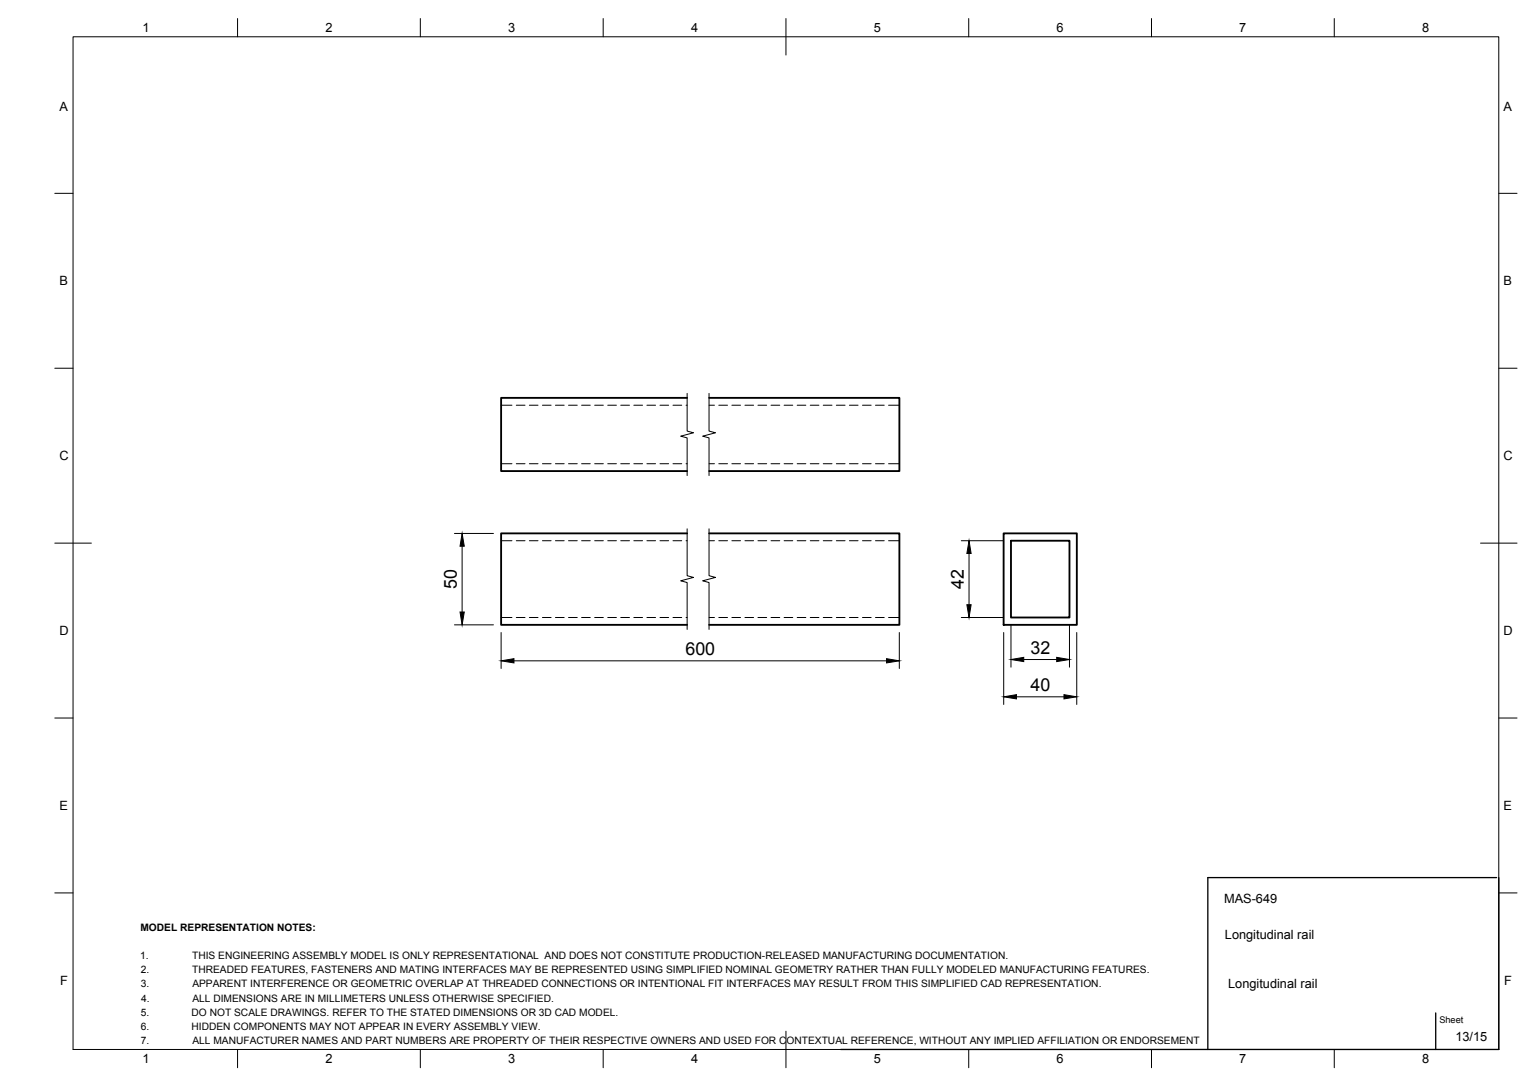
ISO-10303-21;
HEADER;
/* Generated by software containing ST-Developer
 * from STEP Tools, Inc. (www.steptools.com) 
 */

FILE_DESCRIPTION(
/* description */ ('Independent equipment support assembly with bolted 600 x 500 mm welde
d perimeter frame, four adjustable legs and swivel feet. Nominal overa
ll height 518 mm. No load rating assigned.'),
/* implementation_level */ '2;1');

FILE_NAME(
/* name */ 'Longitudinal rail.step',
/* time_stamp */ '2026-11-07T17:30:39-08:00',
/* author */ (''),
/* organization */ (''),
/* preprocessor_version */ 'ST-DEVELOPER v20.2',
/* originating_system */ 'Autodesk Translation Framework v15.17.0.0',
/* authorisation */ '');

FILE_SCHEMA (('AUTOMOTIVE_DESIGN { 1 0 10303 214 3 1 1 }'));
ENDSEC;

DATA;
#10=MECHANICAL_DESIGN_GEOMETRIC_PRESENTATION_REPRESENTATION('',(#2208),#63755);
#2176=SHAPE_REPRESENTATION_RELATIONSHIP('SRR','None',#63860,#2192);
#2192=ADVANCED_BREP_SHAPE_REPRESENTATION('',(#2224),#63738);
#2208=STYLED_ITEM('',(#63958),#2224);
#2224=MANIFOLD_SOLID_BREP('Body1',#14309);
#2240=FACE_BOUND('',#3072,.T.);
#2241=FACE_BOUND('',#3074,.T.);
#2303=FACE_OUTER_BOUND('',#3063,.T.);
#2304=FACE_OUTER_BOUND('',#3064,.T.);
#2305=FACE_OUTER_BOUND('',#3065,.T.);
#2306=FACE_OUTER_BOUND('',#3066,.T.);
#2307=FACE_OUTER_BOUND('',#3067,.T.);
#2308=FACE_OUTER_BOUND('',#3068,.T.);
#2309=FACE_OUTER_BOUND('',#3069,.T.);
#2310=FACE_OUTER_BOUND('',#3070,.T.);
#2311=FACE_OUTER_BOUND('',#3071,.T.);
#2312=FACE_OUTER_BOUND('',#3073,.T.);
#3063=EDGE_LOOP('',(#9127,#9128,#9129,#9130));
#3064=EDGE_LOOP('',(#9131,#9132,#9133,#9134));
#3065=EDGE_LOOP('',(#9135,#9136,#9137,#9138));
#3066=EDGE_LOOP('',(#9139,#9140,#9141,#9142));
#3067=EDGE_LOOP('',(#9143,#9144,#9145,#9146));
#3068=EDGE_LOOP('',(#9147,#9148,#9149,#9150));
#3069=EDGE_LOOP('',(#9151,#9152,#9153,#9154));
#3070=EDGE_LOOP('',(#9155,#9156,#9157,#9158));
#3071=EDGE_LOOP('',(#9159,#9160,#9161,#9162));
#3072=EDGE_LOOP('',(#9163,#9164,#9165,#9166));
#3073=EDGE_LOOP('',(#9167,#9168,#9169,#9170));
#3074=EDGE_LOOP('',(#9171,#9172,#9173,#9174));
#3886=LINE('',#18383,#4722);
#3887=LINE('',#18385,#4723);
#3888=LINE('',#18387,#4724);
#3889=LINE('',#18388,#4725);
#3890=LINE('',#18391,#4726);
#3891=LINE('',#18393,#4727);
#3892=LINE('',#18394,#4728);
#3893=LINE('',#18397,#4729);
#3894=LINE('',#18399,#4730);
#3895=LINE('',#18400,#4731);
#3896=LINE('',#18402,#4732);
#3897=LINE('',#18403,#4733);
#3898=LINE('',#18407,#4734);
#3899=LINE('',#18409,#4735);
#3900=LINE('',#18411,#4736);
#3901=LINE('',#18412,#4737);
#3902=LINE('',#18415,#4738);
#3903=LINE('',#18417,#4739);
#3904=LINE('',#18418,#4740);
#3905=LINE('',#18421,#4741);
#3906=LINE('',#18423,#4742);
#3907=LINE('',#18424,#4743);
#3908=LINE('',#18426,#4744);
#3909=LINE('',#18427,#4745);
#4722=VECTOR('',#15523,10.);
#4723=VECTOR('',#15524,10.);
#4724=VECTOR('',#15525,10.);
#4725=VECTOR('',#15526,10.);
#4726=VECTOR('',#15529,10.);
#4727=VECTOR('',#15530,10.);
#4728=VECTOR('',#15531,10.);
#4729=VECTOR('',#15534,10.);
#4730=VECTOR('',#15535,10.);
#4731=VECTOR('',#15536,10.);
#4732=VECTOR('',#15539,10.);
#4733=VECTOR('',#15540,10.);
#4734=VECTOR('',#15543,10.);
#4735=VECTOR('',#15544,10.);
#4736=VECTOR('',#15545,10.);
#4737=VECTOR('',#15546,10.);
#4738=VECTOR('',#15549,10.);
#4739=VECTOR('',#15550,10.);
#4740=VECTOR('',#15551,10.);
#4741=VECTOR('',#15554,10.);
#4742=VECTOR('',#15555,10.);
#4743=VECTOR('',#15556,10.);
#4744=VECTOR('',#15559,10.);
#4745=VECTOR('',#15560,10.);
#5558=VERTEX_POINT('',#18381);
#5559=VERTEX_POINT('',#18382);
#5560=VERTEX_POINT('',#18384);
#5561=VERTEX_POINT('',#18386);
#5562=VERTEX_POINT('',#18390);
#5563=VERTEX_POINT('',#18392);
#5564=VERTEX_POINT('',#18396);
#5565=VERTEX_POINT('',#18398);
#5566=VERTEX_POINT('',#18405);
#5567=VERTEX_POINT('',#18406);
#5568=VERTEX_POINT('',#18408);
#5569=VERTEX_POINT('',#18410);
#5570=VERTEX_POINT('',#18414);
#5571=VERTEX_POINT('',#18416);
#5572=VERTEX_POINT('',#18420);
#5573=VERTEX_POINT('',#18422);
#6986=EDGE_CURVE('',#5558,#5559,#3886,.T.);
#6987=EDGE_CURVE('',#5559,#5560,#3887,.T.);
#6988=EDGE_CURVE('',#5561,#5560,#3888,.T.);
#6989=EDGE_CURVE('',#5558,#5561,#3889,.T.);
#6990=EDGE_CURVE('',#5562,#5558,#3890,.T.);
#6991=EDGE_CURVE('',#5563,#5561,#3891,.T.);
#6992=EDGE_CURVE('',#5562,#5563,#3892,.T.);
#6993=EDGE_CURVE('',#5564,#5562,#3893,.T.);
#6994=EDGE_CURVE('',#5565,#5563,#3894,.T.);
#6995=EDGE_CURVE('',#5564,#5565,#3895,.T.);
#6996=EDGE_CURVE('',#5559,#5564,#3896,.T.);
#6997=EDGE_CURVE('',#5560,#5565,#3897,.T.);
#6998=EDGE_CURVE('',#5566,#5567,#3898,.T.);
#6999=EDGE_CURVE('',#5567,#5568,#3899,.T.);
#7000=EDGE_CURVE('',#5569,#5568,#3900,.T.);
#7001=EDGE_CURVE('',#5566,#5569,#3901,.T.);
#7002=EDGE_CURVE('',#5570,#5566,#3902,.T.);
#7003=EDGE_CURVE('',#5571,#5569,#3903,.T.);
#7004=EDGE_CURVE('',#5570,#5571,#3904,.T.);
#7005=EDGE_CURVE('',#5572,#5570,#3905,.T.);
#7006=EDGE_CURVE('',#5573,#5571,#3906,.T.);
#7007=EDGE_CURVE('',#5572,#5573,#3907,.T.);
#7008=EDGE_CURVE('',#5567,#5572,#3908,.T.);
#7009=EDGE_CURVE('',#5568,#5573,#3909,.T.);
#9127=ORIENTED_EDGE('',*,*,#6986,.T.);
#9128=ORIENTED_EDGE('',*,*,#6987,.T.);
#9129=ORIENTED_EDGE('',*,*,#6988,.F.);
#9130=ORIENTED_EDGE('',*,*,#6989,.F.);
#9131=ORIENTED_EDGE('',*,*,#6990,.T.);
#9132=ORIENTED_EDGE('',*,*,#6989,.T.);
#9133=ORIENTED_EDGE('',*,*,#6991,.F.);
#9134=ORIENTED_EDGE('',*,*,#6992,.F.);
#9135=ORIENTED_EDGE('',*,*,#6993,.T.);
#9136=ORIENTED_EDGE('',*,*,#6992,.T.);
#9137=ORIENTED_EDGE('',*,*,#6994,.F.);
#9138=ORIENTED_EDGE('',*,*,#6995,.F.);
#9139=ORIENTED_EDGE('',*,*,#6996,.T.);
#9140=ORIENTED_EDGE('',*,*,#6995,.T.);
#9141=ORIENTED_EDGE('',*,*,#6997,.F.);
#9142=ORIENTED_EDGE('',*,*,#6987,.F.);
#9143=ORIENTED_EDGE('',*,*,#6998,.T.);
#9144=ORIENTED_EDGE('',*,*,#6999,.T.);
#9145=ORIENTED_EDGE('',*,*,#7000,.F.);
#9146=ORIENTED_EDGE('',*,*,#7001,.F.);
#9147=ORIENTED_EDGE('',*,*,#7002,.T.);
#9148=ORIENTED_EDGE('',*,*,#7001,.T.);
#9149=ORIENTED_EDGE('',*,*,#7003,.F.);
#9150=ORIENTED_EDGE('',*,*,#7004,.F.);
#9151=ORIENTED_EDGE('',*,*,#7005,.T.);
#9152=ORIENTED_EDGE('',*,*,#7004,.T.);
#9153=ORIENTED_EDGE('',*,*,#7006,.F.);
#9154=ORIENTED_EDGE('',*,*,#7007,.F.);
#9155=ORIENTED_EDGE('',*,*,#7008,.T.);
#9156=ORIENTED_EDGE('',*,*,#7007,.T.);
#9157=ORIENTED_EDGE('',*,*,#7009,.F.);
#9158=ORIENTED_EDGE('',*,*,#6999,.F.);
#9159=ORIENTED_EDGE('',*,*,#7009,.T.);
#9160=ORIENTED_EDGE('',*,*,#7006,.T.);
#9161=ORIENTED_EDGE('',*,*,#7003,.T.);
#9162=ORIENTED_EDGE('',*,*,#7000,.T.);
#9163=ORIENTED_EDGE('',*,*,#6997,.T.);
#9164=ORIENTED_EDGE('',*,*,#6994,.T.);
#9165=ORIENTED_EDGE('',*,*,#6991,.T.);
#9166=ORIENTED_EDGE('',*,*,#6988,.T.);
#9167=ORIENTED_EDGE('',*,*,#7008,.F.);
#9168=ORIENTED_EDGE('',*,*,#6998,.F.);
#9169=ORIENTED_EDGE('',*,*,#7002,.F.);
#9170=ORIENTED_EDGE('',*,*,#7005,.F.);
#9171=ORIENTED_EDGE('',*,*,#6996,.F.);
#9172=ORIENTED_EDGE('',*,*,#6986,.F.);
#9173=ORIENTED_EDGE('',*,*,#6990,.F.);
#9174=ORIENTED_EDGE('',*,*,#6993,.F.);
#13409=PLANE('',#14505);
#13410=PLANE('',#14506);
#13411=PLANE('',#14507);
#13412=PLANE('',#14508);
#13413=PLANE('',#14509);
#13414=PLANE('',#14510);
#13415=PLANE('',#14511);
#13416=PLANE('',#14512);
#13417=PLANE('',#14513);
#13418=PLANE('',#14514);
#13549=ADVANCED_FACE('',(#2303),#13409,.T.);
#13550=ADVANCED_FACE('',(#2304),#13410,.T.);
#13551=ADVANCED_FACE('',(#2305),#13411,.T.);
#13552=ADVANCED_FACE('',(#2306),#13412,.T.);
#13553=ADVANCED_FACE('',(#2307),#13413,.T.);
#13554=ADVANCED_FACE('',(#2308),#13414,.T.);
#13555=ADVANCED_FACE('',(#2309),#13415,.T.);
#13556=ADVANCED_FACE('',(#2310),#13416,.T.);
#13557=ADVANCED_FACE('',(#2311,#2240),#13417,.T.);
#13558=ADVANCED_FACE('',(#2312,#2241),#13418,.F.);
#14309=CLOSED_SHELL('',(#13549,#13550,#13551,#13552,#13553,#13554,#13555,
#13556,#13557,#13558));
#14504=AXIS2_PLACEMENT_3D('',#18379,#15519,#15520);
#14505=AXIS2_PLACEMENT_3D('',#18380,#15521,#15522);
#14506=AXIS2_PLACEMENT_3D('',#18389,#15527,#15528);
#14507=AXIS2_PLACEMENT_3D('',#18395,#15532,#15533);
#14508=AXIS2_PLACEMENT_3D('',#18401,#15537,#15538);
#14509=AXIS2_PLACEMENT_3D('',#18404,#15541,#15542);
#14510=AXIS2_PLACEMENT_3D('',#18413,#15547,#15548);
#14511=AXIS2_PLACEMENT_3D('',#18419,#15552,#15553);
#14512=AXIS2_PLACEMENT_3D('',#18425,#15557,#15558);
#14513=AXIS2_PLACEMENT_3D('',#18428,#15561,#15562);
#14514=AXIS2_PLACEMENT_3D('',#18429,#15563,#15564);
#15519=DIRECTION('axis',(0.,0.,1.));
#15520=DIRECTION('refdir',(1.,0.,0.));
#15521=DIRECTION('center_axis',(0.,1.,0.));
#15522=DIRECTION('ref_axis',(-1.,0.,0.));
#15523=DIRECTION('',(-1.,0.,0.));
#15524=DIRECTION('',(0.,0.,1.));
#15525=DIRECTION('',(-1.,0.,0.));
#15526=DIRECTION('',(0.,0.,1.));
#15527=DIRECTION('center_axis',(-1.,0.,0.));
#15528=DIRECTION('ref_axis',(0.,-1.,0.));
#15529=DIRECTION('',(0.,-1.,0.));
#15530=DIRECTION('',(0.,-1.,0.));
#15531=DIRECTION('',(0.,0.,1.));
#15532=DIRECTION('center_axis',(0.,-1.,0.));
#15533=DIRECTION('ref_axis',(1.,0.,0.));
#15534=DIRECTION('',(1.,0.,0.));
#15535=DIRECTION('',(1.,0.,0.));
#15536=DIRECTION('',(0.,0.,1.));
#15537=DIRECTION('center_axis',(1.,0.,0.));
#15538=DIRECTION('ref_axis',(0.,1.,0.));
#15539=DIRECTION('',(0.,1.,0.));
#15540=DIRECTION('',(0.,1.,0.));
#15541=DIRECTION('center_axis',(0.,1.,0.));
#15542=DIRECTION('ref_axis',(-1.,0.,0.));
#15543=DIRECTION('',(-1.,0.,0.));
#15544=DIRECTION('',(0.,0.,1.));
#15545=DIRECTION('',(-1.,0.,0.));
#15546=DIRECTION('',(0.,0.,1.));
#15547=DIRECTION('center_axis',(1.,0.,0.));
#15548=DIRECTION('ref_axis',(0.,1.,0.));
#15549=DIRECTION('',(0.,1.,0.));
#15550=DIRECTION('',(0.,1.,0.));
#15551=DIRECTION('',(0.,0.,1.));
#15552=DIRECTION('center_axis',(0.,-1.,0.));
#15553=DIRECTION('ref_axis',(1.,0.,0.));
#15554=DIRECTION('',(1.,0.,0.));
#15555=DIRECTION('',(1.,0.,0.));
#15556=DIRECTION('',(0.,0.,1.));
#15557=DIRECTION('center_axis',(-1.,0.,0.));
#15558=DIRECTION('ref_axis',(0.,-1.,0.));
#15559=DIRECTION('',(0.,-1.,0.));
#15560=DIRECTION('',(0.,-1.,0.));
#15561=DIRECTION('center_axis',(0.,0.,1.));
#15562=DIRECTION('ref_axis',(1.,0.,0.));
#15563=DIRECTION('center_axis',(0.,0.,1.));
#15564=DIRECTION('ref_axis',(1.,0.,0.));
#18379=CARTESIAN_POINT('',(0.,0.,0.));
#18380=CARTESIAN_POINT('Origin',(16.,-21.,0.));
#18381=CARTESIAN_POINT('',(16.,-21.,0.));
#18382=CARTESIAN_POINT('',(-16.,-21.,0.));
#18383=CARTESIAN_POINT('',(-16.,-21.,0.));
#18384=CARTESIAN_POINT('',(-16.,-21.,600.));
#18385=CARTESIAN_POINT('',(-16.,-21.,0.));
#18386=CARTESIAN_POINT('',(16.,-21.,600.));
#18387=CARTESIAN_POINT('',(-16.,-21.,600.));
#18388=CARTESIAN_POINT('',(16.,-21.,0.));
#18389=CARTESIAN_POINT('Origin',(16.,21.,0.));
#18390=CARTESIAN_POINT('',(16.,21.,0.));
#18391=CARTESIAN_POINT('',(16.,-21.,0.));
#18392=CARTESIAN_POINT('',(16.,21.,600.));
#18393=CARTESIAN_POINT('',(16.,-21.,600.));
#18394=CARTESIAN_POINT('',(16.,21.,0.));
#18395=CARTESIAN_POINT('Origin',(-16.,21.,0.));
#18396=CARTESIAN_POINT('',(-16.,21.,0.));
#18397=CARTESIAN_POINT('',(16.,21.,0.));
#18398=CARTESIAN_POINT('',(-16.,21.,600.));
#18399=CARTESIAN_POINT('',(16.,21.,600.));
#18400=CARTESIAN_POINT('',(-16.,21.,0.));
#18401=CARTESIAN_POINT('Origin',(-16.,-21.,0.));
#18402=CARTESIAN_POINT('',(-16.,21.,0.));
#18403=CARTESIAN_POINT('',(-16.,21.,600.));
#18404=CARTESIAN_POINT('Origin',(20.,25.,0.));
#18405=CARTESIAN_POINT('',(20.,25.,0.));
#18406=CARTESIAN_POINT('',(-20.,25.,0.));
#18407=CARTESIAN_POINT('',(20.,25.,0.));
#18408=CARTESIAN_POINT('',(-20.,25.,600.));
#18409=CARTESIAN_POINT('',(-20.,25.,0.));
#18410=CARTESIAN_POINT('',(20.,25.,600.));
#18411=CARTESIAN_POINT('',(20.,25.,600.));
#18412=CARTESIAN_POINT('',(20.,25.,0.));
#18413=CARTESIAN_POINT('Origin',(20.,-25.,0.));
#18414=CARTESIAN_POINT('',(20.,-25.,0.));
#18415=CARTESIAN_POINT('',(20.,-25.,0.));
#18416=CARTESIAN_POINT('',(20.,-25.,600.));
#18417=CARTESIAN_POINT('',(20.,-25.,600.));
#18418=CARTESIAN_POINT('',(20.,-25.,0.));
#18419=CARTESIAN_POINT('Origin',(-20.,-25.,0.));
#18420=CARTESIAN_POINT('',(-20.,-25.,0.));
#18421=CARTESIAN_POINT('',(-20.,-25.,0.));
#18422=CARTESIAN_POINT('',(-20.,-25.,600.));
#18423=CARTESIAN_POINT('',(-20.,-25.,600.));
#18424=CARTESIAN_POINT('',(-20.,-25.,0.));
#18425=CARTESIAN_POINT('Origin',(-20.,25.,0.));
#18426=CARTESIAN_POINT('',(-20.,25.,0.));
#18427=CARTESIAN_POINT('',(-20.,25.,600.));
#18428=CARTESIAN_POINT('Origin',(0.,0.,600.));
#18429=CARTESIAN_POINT('Origin',(0.,0.,0.));
#63718=UNCERTAINTY_MEASURE_WITH_UNIT(LENGTH_MEASURE(0.01),#63756,
'DISTANCE_ACCURACY_VALUE',
'Maximum model space distance between geometric entities at asserted c
onnectivities');
#63735=UNCERTAINTY_MEASURE_WITH_UNIT(LENGTH_MEASURE(0.01),#63756,
'DISTANCE_ACCURACY_VALUE',
'Maximum model space distance between geometric entities at asserted c
onnectivities');
#63738=(
GEOMETRIC_REPRESENTATION_CONTEXT(3)
GLOBAL_UNCERTAINTY_ASSIGNED_CONTEXT((#63718))
GLOBAL_UNIT_ASSIGNED_CONTEXT((#63756,#63758,#63759))
REPRESENTATION_CONTEXT('','3D')
);
#63755=(
GEOMETRIC_REPRESENTATION_CONTEXT(3)
GLOBAL_UNCERTAINTY_ASSIGNED_CONTEXT((#63735))
GLOBAL_UNIT_ASSIGNED_CONTEXT((#63756,#63758,#63759))
REPRESENTATION_CONTEXT('','3D')
);
#63756=(
LENGTH_UNIT()
NAMED_UNIT(*)
SI_UNIT(.MILLI.,.METRE.)
);
#63758=(
NAMED_UNIT(*)
PLANE_ANGLE_UNIT()
SI_UNIT($,.RADIAN.)
);
#63759=(
NAMED_UNIT(*)
SI_UNIT($,.STERADIAN.)
SOLID_ANGLE_UNIT()
);
#63762=SHAPE_DEFINITION_REPRESENTATION(#63781,#63860);
#63781=PRODUCT_DEFINITION_SHAPE('',$,#63880);
#63860=SHAPE_REPRESENTATION('',(#14504),#63738);
#63877=PRODUCT_DEFINITION_CONTEXT('part definition',#63936,'design');
#63880=PRODUCT_DEFINITION('Longitudinal rail','Longitudinal rail',#63899,
#63877);
#63899=PRODUCT_DEFINITION_FORMATION('',$,#63940);
#63936=APPLICATION_CONTEXT(
'Core Data for Automotive Mechanical Design Process');
#63937=PRODUCT_CONTEXT('part definition',#63936,'mechanical');
#63940=PRODUCT('Longitudinal rail','Longitudinal rail',
'Steel rectangular hollow section, 50 x 40 mm, 4 mm wall. Square cut e
nds; weld to adjoining rails and corner plates.',(#63937));
#63958=PRESENTATION_STYLE_ASSIGNMENT((#63965));
#63965=SURFACE_STYLE_USAGE(.BOTH.,#63972);
#63972=SURFACE_SIDE_STYLE('',(#63979));
#63979=SURFACE_STYLE_FILL_AREA(#63986);
#63986=FILL_AREA_STYLE('Dark blue',(#63993));
#63993=FILL_AREA_STYLE_COLOUR('Dark blue',#64000);
#64000=COLOUR_RGB('Dark blue',0.0901960784313725,0.270588235294118,0.513725490196078);
ENDSEC;
END-ISO-10303-21;
